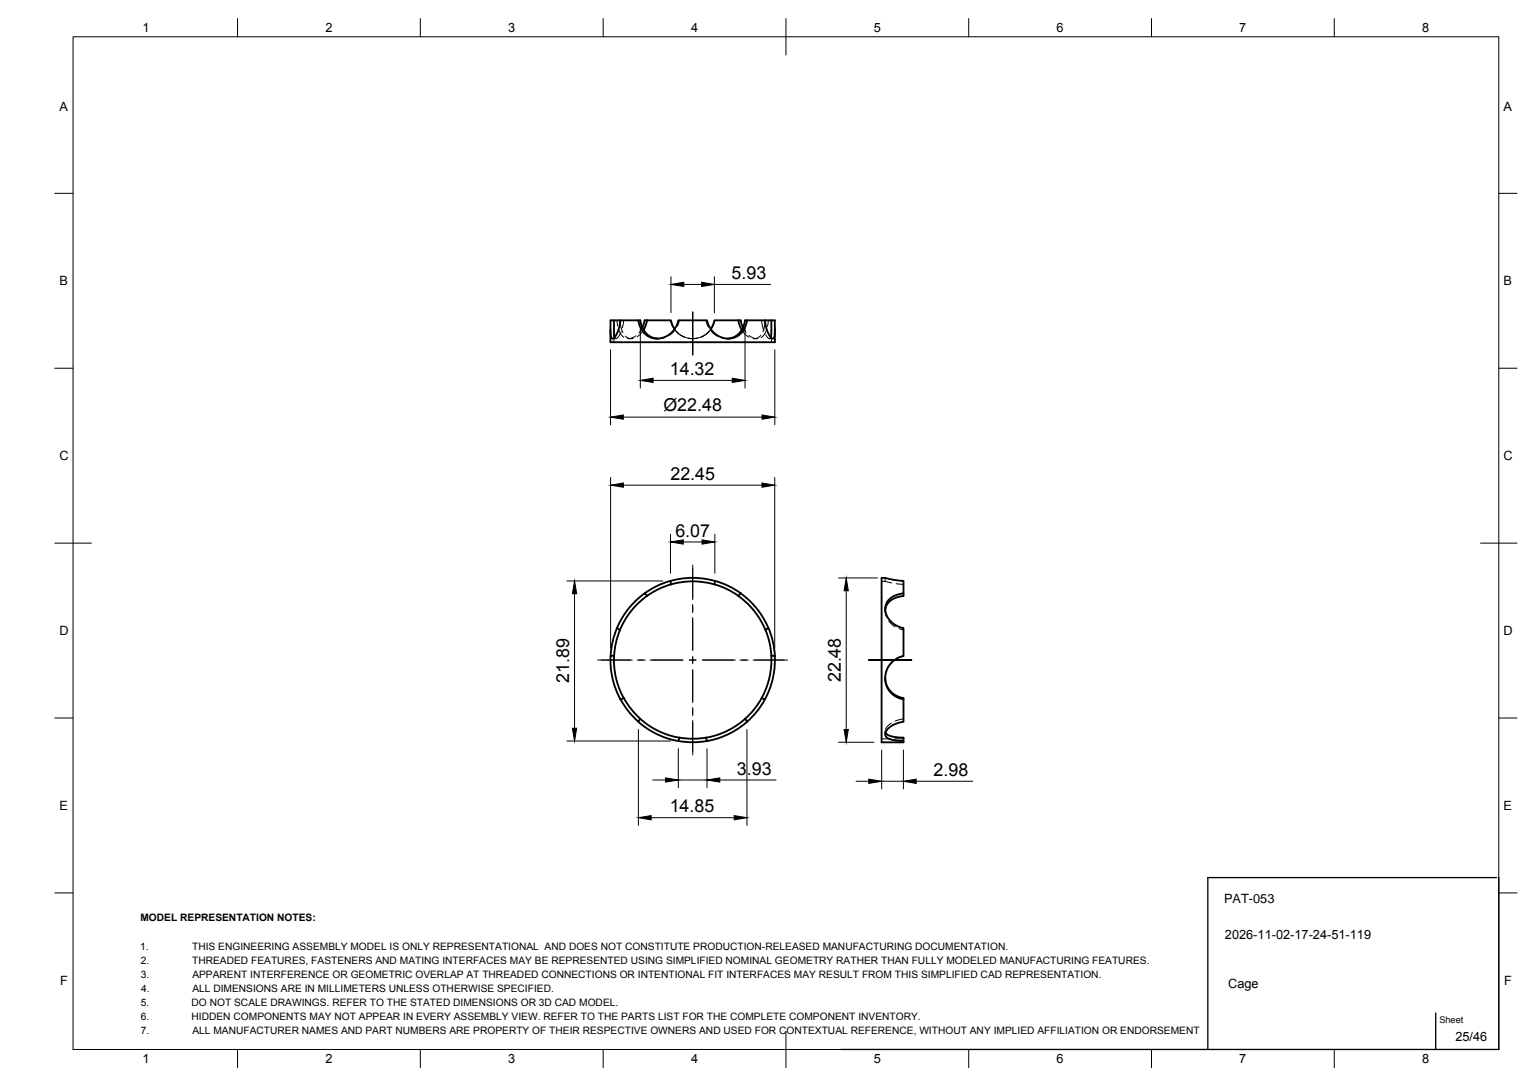
ISO-10303-21;
HEADER;
/* Generated by software containing ST-Developer
 * from STEP Tools, Inc. (www.steptools.com) 
 */

FILE_DESCRIPTION(
/* description */ ('Hand-operated arbor press'),
/* implementation_level */ '2;1');

FILE_NAME(
/* name */ 'Cage.step',
/* time_stamp */ '2026-10-28T03:25:25-07:00',
/* author */ (''),
/* organization */ (''),
/* preprocessor_version */ 'ST-DEVELOPER v20.2',
/* originating_system */ 'Autodesk Translation Framework v15.17.0.0',
/* authorisation */ '');

FILE_SCHEMA (('AUTOMOTIVE_DESIGN { 1 0 10303 214 3 1 1 }'));
ENDSEC;

DATA;
#10=MECHANICAL_DESIGN_GEOMETRIC_PRESENTATION_REPRESENTATION('',(#611),#32751);
#439=B_SPLINE_CURVE_WITH_KNOTS('',3,(#18826,#18827,#18828,#18829,#18830,
#18831,#18832,#18833,#18834,#18835,#18836,#18837,#18838,#18839,#18840,#18841,
#18842,#18843,#18844,#18845,#18846,#18847),.UNSPECIFIED.,.F.,.F.,(4,2,2,
2,2,2,2,2,2,2,4),(0.0591825211272536,0.157966726598481,0.236950089897721,
0.315933453196962,0.391576304923761,0.46721915665056,0.54286200837736,0.618504860104159,
0.697488223403399,0.77647158670264,0.875255792173867),.UNSPECIFIED.);
#440=B_SPLINE_CURVE_WITH_KNOTS('',3,(#18851,#18852,#18853,#18854,#18855,
#18856,#18857,#18858,#18859,#18860,#18861,#18862,#18863,#18864,#18865,#18866,
#18867,#18868,#18869,#18870,#18871,#18872),.UNSPECIFIED.,.F.,.F.,(4,2,2,
2,2,2,2,2,2,2,4),(0.0581119756758434,0.106553146291161,0.213106292582322,
0.30849933801665,0.386091982889075,0.4636846277615,0.541277272633925,0.61886991750635,
0.714262962940678,0.820816109231839,0.869257279847157),.UNSPECIFIED.);
#441=B_SPLINE_CURVE_WITH_KNOTS('',3,(#18878,#18879,#18880,#18881,#18882,
#18883,#18884,#18885,#18886,#18887,#18888,#18889,#18890,#18891,#18892,#18893,
#18894,#18895,#18896,#18897,#18898,#18899),.UNSPECIFIED.,.F.,.F.,(4,2,2,
2,2,2,2,2,2,2,4),(0.0581119756758434,0.106553146291161,0.213106292582322,
0.30849933801665,0.386091982889075,0.4636846277615,0.541277272633925,0.61886991750635,
0.714262962940679,0.820816109231839,0.869257279847157),.UNSPECIFIED.);
#442=B_SPLINE_CURVE_WITH_KNOTS('',3,(#18903,#18904,#18905,#18906,#18907,
#18908,#18909,#18910,#18911,#18912,#18913,#18914,#18915,#18916,#18917,#18918,
#18919,#18920,#18921,#18922,#18923,#18924),.UNSPECIFIED.,.F.,.F.,(4,2,2,
2,2,2,2,2,2,2,4),(0.0581119756758433,0.106553146291161,0.213106292582322,
0.308499338016649,0.386091982889075,0.4636846277615,0.541277272633925,0.61886991750635,
0.714262962940678,0.820816109231839,0.869257279847157),.UNSPECIFIED.);
#443=B_SPLINE_CURVE_WITH_KNOTS('',3,(#18933,#18934,#18935,#18936,#18937,
#18938,#18939,#18940,#18941,#18942,#18943,#18944,#18945,#18946,#18947,#18948,
#18949,#18950,#18951,#18952,#18953,#18954),.UNSPECIFIED.,.F.,.F.,(4,2,2,
2,2,2,2,2,2,2,4),(0.0581119756758433,0.106553146291161,0.213106292582322,
0.30849933801665,0.386091982889075,0.4636846277615,0.541277272633925,0.61886991750635,
0.714262962940678,0.820816109231839,0.869257279847157),.UNSPECIFIED.);
#444=B_SPLINE_CURVE_WITH_KNOTS('',3,(#18958,#18959,#18960,#18961,#18962,
#18963,#18964,#18965,#18966,#18967,#18968,#18969,#18970,#18971,#18972,#18973,
#18974,#18975,#18976,#18977,#18978,#18979),.UNSPECIFIED.,.F.,.F.,(4,2,2,
2,2,2,2,2,2,2,4),(0.0581119756758434,0.106553146291161,0.213106292582322,
0.30849933801665,0.386091982889075,0.4636846277615,0.541277272633925,0.61886991750635,
0.714262962940678,0.820816109231839,0.869257279847157),.UNSPECIFIED.);
#445=B_SPLINE_CURVE_WITH_KNOTS('',3,(#18983,#18984,#18985,#18986,#18987,
#18988,#18989,#18990,#18991,#18992,#18993,#18994,#18995,#18996,#18997,#18998,
#18999,#19000,#19001,#19002,#19003,#19004),.UNSPECIFIED.,.F.,.F.,(4,2,2,
2,2,2,2,2,2,2,4),(0.0581119756758434,0.106553146291161,0.213106292582322,
0.30849933801665,0.386091982889075,0.4636846277615,0.541277272633925,0.61886991750635,
0.714262962940678,0.820816109231839,0.869257279847157),.UNSPECIFIED.);
#446=B_SPLINE_CURVE_WITH_KNOTS('',3,(#19008,#19009,#19010,#19011,#19012,
#19013,#19014,#19015,#19016,#19017,#19018,#19019,#19020,#19021,#19022,#19023,
#19024,#19025,#19026,#19027,#19028,#19029),.UNSPECIFIED.,.F.,.F.,(4,2,2,
2,2,2,2,2,2,2,4),(0.0581119756758433,0.106553146291161,0.213106292582322,
0.30849933801665,0.386091982889075,0.4636846277615,0.541277272633925,0.61886991750635,
0.714262962940678,0.820816109231839,0.869257279847157),.UNSPECIFIED.);
#447=B_SPLINE_CURVE_WITH_KNOTS('',3,(#19037,#19038,#19039,#19040,#19041,
#19042,#19043,#19044,#19045,#19046,#19047,#19048,#19049,#19050,#19051,#19052,
#19053,#19054,#19055,#19056,#19057,#19058),.UNSPECIFIED.,.F.,.F.,(4,2,2,
2,2,2,2,2,2,2,4),(0.0591825211272536,0.157966726598481,0.236950089897721,
0.315933453196962,0.391576304923761,0.467219156650561,0.54286200837736,
0.618504860104159,0.697488223403399,0.77647158670264,0.875255792173867),
 .UNSPECIFIED.);
#448=B_SPLINE_CURVE_WITH_KNOTS('',3,(#19066,#19067,#19068,#19069,#19070,
#19071,#19072,#19073,#19074,#19075,#19076,#19077,#19078,#19079,#19080,#19081,
#19082,#19083,#19084,#19085,#19086,#19087),.UNSPECIFIED.,.F.,.F.,(4,2,2,
2,2,2,2,2,2,2,4),(0.0591825211272536,0.157966726598481,0.236950089897722,
0.315933453196962,0.391576304923761,0.467219156650561,0.54286200837736,
0.618504860104159,0.697488223403399,0.77647158670264,0.875255792173867),
 .UNSPECIFIED.);
#449=B_SPLINE_CURVE_WITH_KNOTS('',3,(#19097,#19098,#19099,#19100,#19101,
#19102,#19103,#19104,#19105,#19106,#19107,#19108,#19109,#19110,#19111,#19112,
#19113,#19114,#19115,#19116,#19117,#19118),.UNSPECIFIED.,.F.,.F.,(4,2,2,
2,2,2,2,2,2,2,4),(0.0591825211272536,0.157966726598481,0.236950089897721,
0.315933453196962,0.391576304923761,0.46721915665056,0.54286200837736,0.618504860104159,
0.697488223403399,0.77647158670264,0.875255792173867),.UNSPECIFIED.);
#450=B_SPLINE_CURVE_WITH_KNOTS('',3,(#19126,#19127,#19128,#19129,#19130,
#19131,#19132,#19133,#19134,#19135,#19136,#19137,#19138,#19139,#19140,#19141,
#19142,#19143,#19144,#19145,#19146,#19147),.UNSPECIFIED.,.F.,.F.,(4,2,2,
2,2,2,2,2,2,2,4),(0.0591825211272536,0.157966726598481,0.236950089897721,
0.315933453196962,0.391576304923761,0.46721915665056,0.542862008377359,
0.618504860104159,0.697488223403399,0.776471586702639,0.875255792173867),
 .UNSPECIFIED.);
#451=B_SPLINE_CURVE_WITH_KNOTS('',3,(#19155,#19156,#19157,#19158,#19159,
#19160,#19161,#19162,#19163,#19164,#19165,#19166,#19167,#19168,#19169,#19170,
#19171,#19172,#19173,#19174,#19175,#19176),.UNSPECIFIED.,.F.,.F.,(4,2,2,
2,2,2,2,2,2,2,4),(0.0591825211272536,0.157966726598481,0.236950089897721,
0.315933453196962,0.391576304923761,0.46721915665056,0.54286200837736,0.618504860104159,
0.697488223403399,0.77647158670264,0.875255792173867),.UNSPECIFIED.);
#452=B_SPLINE_CURVE_WITH_KNOTS('',3,(#19185,#19186,#19187,#19188,#19189,
#19190,#19191,#19192,#19193,#19194,#19195,#19196,#19197,#19198,#19199,#19200,
#19201,#19202,#19203,#19204,#19205,#19206),.UNSPECIFIED.,.F.,.F.,(4,2,2,
2,2,2,2,2,2,2,4),(0.0591825211272536,0.157966726598481,0.236950089897721,
0.315933453196962,0.391576304923761,0.46721915665056,0.542862008377359,
0.618504860104159,0.697488223403399,0.776471586702639,0.875255792173867),
 .UNSPECIFIED.);
#464=SPHERICAL_SURFACE('',#13471,0.309556);
#465=SPHERICAL_SURFACE('',#13487,0.309556);
#466=SPHERICAL_SURFACE('',#13492,0.309556);
#467=SPHERICAL_SURFACE('',#13498,0.309556);
#468=SPHERICAL_SURFACE('',#13503,0.309556);
#469=SPHERICAL_SURFACE('',#13508,0.309556);
#470=SPHERICAL_SURFACE('',#13516,0.309556);
#521=SHAPE_REPRESENTATION_RELATIONSHIP('SRR','None',#32951,#563);
#563=ADVANCED_BREP_SHAPE_REPRESENTATION('',(#659),#32725);
#611=STYLED_ITEM('',(#33242),#659);
#659=MANIFOLD_SOLID_BREP('Continuous crown cage',#12509);
#806=FACE_BOUND('',#2358,.T.);
#981=PLANE('',#13484);
#982=PLANE('',#13489);
#983=PLANE('',#13494);
#984=PLANE('',#13500);
#985=PLANE('',#13505);
#986=PLANE('',#13514);
#987=PLANE('',#13518);
#988=PLANE('',#13519);
#1535=FACE_OUTER_BOUND('',#2342,.T.);
#1536=FACE_OUTER_BOUND('',#2343,.T.);
#1537=FACE_OUTER_BOUND('',#2344,.T.);
#1538=FACE_OUTER_BOUND('',#2345,.T.);
#1539=FACE_OUTER_BOUND('',#2346,.T.);
#1540=FACE_OUTER_BOUND('',#2347,.T.);
#1541=FACE_OUTER_BOUND('',#2348,.T.);
#1542=FACE_OUTER_BOUND('',#2349,.T.);
#1543=FACE_OUTER_BOUND('',#2350,.T.);
#1544=FACE_OUTER_BOUND('',#2351,.T.);
#1545=FACE_OUTER_BOUND('',#2352,.T.);
#1546=FACE_OUTER_BOUND('',#2353,.T.);
#1547=FACE_OUTER_BOUND('',#2354,.T.);
#1548=FACE_OUTER_BOUND('',#2355,.T.);
#1549=FACE_OUTER_BOUND('',#2356,.T.);
#1550=FACE_OUTER_BOUND('',#2357,.T.);
#1551=FACE_OUTER_BOUND('',#2359,.T.);
#2342=EDGE_LOOP('',(#9420,#9421,#9422,#9423));
#2343=EDGE_LOOP('',(#9424,#9425,#9426,#9427,#9428,#9429,#9430,#9431,#9432,
#9433,#9434,#9435,#9436,#9437,#9438,#9439,#9440,#9441));
#2344=EDGE_LOOP('',(#9442,#9443,#9444,#9445));
#2345=EDGE_LOOP('',(#9446,#9447,#9448,#9449));
#2346=EDGE_LOOP('',(#9450,#9451,#9452,#9453));
#2347=EDGE_LOOP('',(#9454,#9455,#9456,#9457));
#2348=EDGE_LOOP('',(#9458,#9459,#9460,#9461,#9462,#9463));
#2349=EDGE_LOOP('',(#9464,#9465,#9466,#9467));
#2350=EDGE_LOOP('',(#9468,#9469,#9470,#9471));
#2351=EDGE_LOOP('',(#9472,#9473,#9474,#9475));
#2352=EDGE_LOOP('',(#9476,#9477,#9478,#9479));
#2353=EDGE_LOOP('',(#9480,#9481,#9482,#9483));
#2354=EDGE_LOOP('',(#9484,#9485,#9486,#9487,#9488,#9489,#9490,#9491,#9492,
#9493,#9494,#9495,#9496,#9497,#9498,#9499,#9500,#9501));
#2355=EDGE_LOOP('',(#9502,#9503,#9504,#9505));
#2356=EDGE_LOOP('',(#9506,#9507,#9508,#9509));
#2357=EDGE_LOOP('',(#9510));
#2358=EDGE_LOOP('',(#9511));
#2359=EDGE_LOOP('',(#9512,#9513,#9514,#9515));
#3165=LINE('',#18928,#4336);
#3166=LINE('',#19181,#4337);
#4336=VECTOR('',#15454,1.123812);
#4337=VECTOR('',#15523,1.076188);
#5373=CIRCLE('',#13472,0.303778037777585);
#5374=CIRCLE('',#13473,0.303778037777585);
#5375=CIRCLE('',#13475,1.123812);
#5376=CIRCLE('',#13476,1.123812);
#5377=CIRCLE('',#13477,1.123812);
#5378=CIRCLE('',#13478,1.123812);
#5379=CIRCLE('',#13479,1.123812);
#5380=CIRCLE('',#13480,1.123812);
#5381=CIRCLE('',#13481,1.123812);
#5382=CIRCLE('',#13482,1.123812);
#5383=CIRCLE('',#13483,1.123812);
#5384=CIRCLE('',#13485,1.076188);
#5385=CIRCLE('',#13486,0.303778037777585);
#5386=CIRCLE('',#13488,0.303778037777585);
#5387=CIRCLE('',#13490,1.076188);
#5388=CIRCLE('',#13491,0.303778037777585);
#5389=CIRCLE('',#13493,0.303778037777585);
#5390=CIRCLE('',#13495,1.076188);
#5391=CIRCLE('',#13496,1.076188);
#5392=CIRCLE('',#13497,0.303778037777585);
#5393=CIRCLE('',#13499,0.303778037777585);
#5394=CIRCLE('',#13501,1.076188);
#5395=CIRCLE('',#13502,0.303778037777585);
#5396=CIRCLE('',#13504,0.303778037777585);
#5397=CIRCLE('',#13506,1.076188);
#5398=CIRCLE('',#13507,0.303778037777585);
#5399=CIRCLE('',#13509,0.303778037777585);
#5400=CIRCLE('',#13511,1.076188);
#5401=CIRCLE('',#13512,1.076188);
#5402=CIRCLE('',#13513,1.076188);
#5403=CIRCLE('',#13515,0.303778037777585);
#5404=CIRCLE('',#13517,0.303778037777585);
#5928=VERTEX_POINT('',#18824);
#5929=VERTEX_POINT('',#18825);
#5930=VERTEX_POINT('',#18848);
#5931=VERTEX_POINT('',#18850);
#5932=VERTEX_POINT('',#18875);
#5933=VERTEX_POINT('',#18877);
#5934=VERTEX_POINT('',#18900);
#5935=VERTEX_POINT('',#18902);
#5936=VERTEX_POINT('',#18925);
#5937=VERTEX_POINT('',#18927);
#5938=VERTEX_POINT('',#18930);
#5939=VERTEX_POINT('',#18932);
#5940=VERTEX_POINT('',#18955);
#5941=VERTEX_POINT('',#18957);
#5942=VERTEX_POINT('',#18980);
#5943=VERTEX_POINT('',#18982);
#5944=VERTEX_POINT('',#19005);
#5945=VERTEX_POINT('',#19007);
#5946=VERTEX_POINT('',#19032);
#5947=VERTEX_POINT('',#19036);
#5948=VERTEX_POINT('',#19061);
#5949=VERTEX_POINT('',#19065);
#5950=VERTEX_POINT('',#19090);
#5951=VERTEX_POINT('',#19092);
#5952=VERTEX_POINT('',#19096);
#5953=VERTEX_POINT('',#19121);
#5954=VERTEX_POINT('',#19125);
#5955=VERTEX_POINT('',#19150);
#5956=VERTEX_POINT('',#19154);
#5957=VERTEX_POINT('',#19179);
#5958=VERTEX_POINT('',#19182);
#5959=VERTEX_POINT('',#19184);
#7213=EDGE_CURVE('',#5928,#5929,#439,.T.);
#7214=EDGE_CURVE('',#5930,#5928,#5373,.T.);
#7215=EDGE_CURVE('',#5931,#5930,#440,.T.);
#7216=EDGE_CURVE('',#5929,#5931,#5374,.T.);
#7217=EDGE_CURVE('',#5932,#5930,#5375,.T.);
#7218=EDGE_CURVE('',#5932,#5933,#441,.T.);
#7219=EDGE_CURVE('',#5934,#5933,#5376,.T.);
#7220=EDGE_CURVE('',#5934,#5935,#442,.T.);
#7221=EDGE_CURVE('',#5936,#5935,#5377,.T.);
#7222=EDGE_CURVE('',#5936,#5937,#3165,.T.);
#7223=EDGE_CURVE('',#5937,#5937,#5378,.T.);
#7224=EDGE_CURVE('',#5938,#5936,#5379,.T.);
#7225=EDGE_CURVE('',#5938,#5939,#443,.T.);
#7226=EDGE_CURVE('',#5940,#5939,#5380,.T.);
#7227=EDGE_CURVE('',#5940,#5941,#444,.T.);
#7228=EDGE_CURVE('',#5942,#5941,#5381,.T.);
#7229=EDGE_CURVE('',#5942,#5943,#445,.T.);
#7230=EDGE_CURVE('',#5944,#5943,#5382,.T.);
#7231=EDGE_CURVE('',#5944,#5945,#446,.T.);
#7232=EDGE_CURVE('',#5931,#5945,#5383,.T.);
#7233=EDGE_CURVE('',#5928,#5946,#5384,.T.);
#7234=EDGE_CURVE('',#5946,#5932,#5385,.T.);
#7235=EDGE_CURVE('',#5947,#5946,#447,.T.);
#7236=EDGE_CURVE('',#5933,#5947,#5386,.T.);
#7237=EDGE_CURVE('',#5947,#5948,#5387,.T.);
#7238=EDGE_CURVE('',#5948,#5934,#5388,.T.);
#7239=EDGE_CURVE('',#5949,#5948,#448,.T.);
#7240=EDGE_CURVE('',#5935,#5949,#5389,.T.);
#7241=EDGE_CURVE('',#5949,#5950,#5390,.T.);
#7242=EDGE_CURVE('',#5950,#5951,#5391,.T.);
#7243=EDGE_CURVE('',#5951,#5938,#5392,.T.);
#7244=EDGE_CURVE('',#5952,#5951,#449,.T.);
#7245=EDGE_CURVE('',#5939,#5952,#5393,.T.);
#7246=EDGE_CURVE('',#5952,#5953,#5394,.T.);
#7247=EDGE_CURVE('',#5953,#5940,#5395,.T.);
#7248=EDGE_CURVE('',#5954,#5953,#450,.T.);
#7249=EDGE_CURVE('',#5941,#5954,#5396,.T.);
#7250=EDGE_CURVE('',#5954,#5955,#5397,.T.);
#7251=EDGE_CURVE('',#5955,#5942,#5398,.T.);
#7252=EDGE_CURVE('',#5956,#5955,#451,.T.);
#7253=EDGE_CURVE('',#5943,#5956,#5399,.T.);
#7254=EDGE_CURVE('',#5957,#5957,#5400,.T.);
#7255=EDGE_CURVE('',#5957,#5950,#3166,.T.);
#7256=EDGE_CURVE('',#5958,#5929,#5401,.T.);
#7257=EDGE_CURVE('',#5958,#5959,#452,.T.);
#7258=EDGE_CURVE('',#5956,#5959,#5402,.T.);
#7259=EDGE_CURVE('',#5945,#5958,#5403,.T.);
#7260=EDGE_CURVE('',#5959,#5944,#5404,.T.);
#9420=ORIENTED_EDGE('',*,*,#7213,.F.);
#9421=ORIENTED_EDGE('',*,*,#7214,.F.);
#9422=ORIENTED_EDGE('',*,*,#7215,.F.);
#9423=ORIENTED_EDGE('',*,*,#7216,.F.);
#9424=ORIENTED_EDGE('',*,*,#7215,.T.);
#9425=ORIENTED_EDGE('',*,*,#7217,.F.);
#9426=ORIENTED_EDGE('',*,*,#7218,.T.);
#9427=ORIENTED_EDGE('',*,*,#7219,.F.);
#9428=ORIENTED_EDGE('',*,*,#7220,.T.);
#9429=ORIENTED_EDGE('',*,*,#7221,.F.);
#9430=ORIENTED_EDGE('',*,*,#7222,.T.);
#9431=ORIENTED_EDGE('',*,*,#7223,.F.);
#9432=ORIENTED_EDGE('',*,*,#7222,.F.);
#9433=ORIENTED_EDGE('',*,*,#7224,.F.);
#9434=ORIENTED_EDGE('',*,*,#7225,.T.);
#9435=ORIENTED_EDGE('',*,*,#7226,.F.);
#9436=ORIENTED_EDGE('',*,*,#7227,.T.);
#9437=ORIENTED_EDGE('',*,*,#7228,.F.);
#9438=ORIENTED_EDGE('',*,*,#7229,.T.);
#9439=ORIENTED_EDGE('',*,*,#7230,.F.);
#9440=ORIENTED_EDGE('',*,*,#7231,.T.);
#9441=ORIENTED_EDGE('',*,*,#7232,.F.);
#9442=ORIENTED_EDGE('',*,*,#7214,.T.);
#9443=ORIENTED_EDGE('',*,*,#7233,.T.);
#9444=ORIENTED_EDGE('',*,*,#7234,.T.);
#9445=ORIENTED_EDGE('',*,*,#7217,.T.);
#9446=ORIENTED_EDGE('',*,*,#7235,.F.);
#9447=ORIENTED_EDGE('',*,*,#7236,.F.);
#9448=ORIENTED_EDGE('',*,*,#7218,.F.);
#9449=ORIENTED_EDGE('',*,*,#7234,.F.);
#9450=ORIENTED_EDGE('',*,*,#7236,.T.);
#9451=ORIENTED_EDGE('',*,*,#7237,.T.);
#9452=ORIENTED_EDGE('',*,*,#7238,.T.);
#9453=ORIENTED_EDGE('',*,*,#7219,.T.);
#9454=ORIENTED_EDGE('',*,*,#7239,.F.);
#9455=ORIENTED_EDGE('',*,*,#7240,.F.);
#9456=ORIENTED_EDGE('',*,*,#7220,.F.);
#9457=ORIENTED_EDGE('',*,*,#7238,.F.);
#9458=ORIENTED_EDGE('',*,*,#7240,.T.);
#9459=ORIENTED_EDGE('',*,*,#7241,.T.);
#9460=ORIENTED_EDGE('',*,*,#7242,.T.);
#9461=ORIENTED_EDGE('',*,*,#7243,.T.);
#9462=ORIENTED_EDGE('',*,*,#7224,.T.);
#9463=ORIENTED_EDGE('',*,*,#7221,.T.);
#9464=ORIENTED_EDGE('',*,*,#7244,.F.);
#9465=ORIENTED_EDGE('',*,*,#7245,.F.);
#9466=ORIENTED_EDGE('',*,*,#7225,.F.);
#9467=ORIENTED_EDGE('',*,*,#7243,.F.);
#9468=ORIENTED_EDGE('',*,*,#7245,.T.);
#9469=ORIENTED_EDGE('',*,*,#7246,.T.);
#9470=ORIENTED_EDGE('',*,*,#7247,.T.);
#9471=ORIENTED_EDGE('',*,*,#7226,.T.);
#9472=ORIENTED_EDGE('',*,*,#7248,.F.);
#9473=ORIENTED_EDGE('',*,*,#7249,.F.);
#9474=ORIENTED_EDGE('',*,*,#7227,.F.);
#9475=ORIENTED_EDGE('',*,*,#7247,.F.);
#9476=ORIENTED_EDGE('',*,*,#7249,.T.);
#9477=ORIENTED_EDGE('',*,*,#7250,.T.);
#9478=ORIENTED_EDGE('',*,*,#7251,.T.);
#9479=ORIENTED_EDGE('',*,*,#7228,.T.);
#9480=ORIENTED_EDGE('',*,*,#7229,.F.);
#9481=ORIENTED_EDGE('',*,*,#7251,.F.);
#9482=ORIENTED_EDGE('',*,*,#7252,.F.);
#9483=ORIENTED_EDGE('',*,*,#7253,.F.);
#9484=ORIENTED_EDGE('',*,*,#7254,.F.);
#9485=ORIENTED_EDGE('',*,*,#7255,.T.);
#9486=ORIENTED_EDGE('',*,*,#7241,.F.);
#9487=ORIENTED_EDGE('',*,*,#7239,.T.);
#9488=ORIENTED_EDGE('',*,*,#7237,.F.);
#9489=ORIENTED_EDGE('',*,*,#7235,.T.);
#9490=ORIENTED_EDGE('',*,*,#7233,.F.);
#9491=ORIENTED_EDGE('',*,*,#7213,.T.);
#9492=ORIENTED_EDGE('',*,*,#7256,.F.);
#9493=ORIENTED_EDGE('',*,*,#7257,.T.);
#9494=ORIENTED_EDGE('',*,*,#7258,.F.);
#9495=ORIENTED_EDGE('',*,*,#7252,.T.);
#9496=ORIENTED_EDGE('',*,*,#7250,.F.);
#9497=ORIENTED_EDGE('',*,*,#7248,.T.);
#9498=ORIENTED_EDGE('',*,*,#7246,.F.);
#9499=ORIENTED_EDGE('',*,*,#7244,.T.);
#9500=ORIENTED_EDGE('',*,*,#7242,.F.);
#9501=ORIENTED_EDGE('',*,*,#7255,.F.);
#9502=ORIENTED_EDGE('',*,*,#7216,.T.);
#9503=ORIENTED_EDGE('',*,*,#7232,.T.);
#9504=ORIENTED_EDGE('',*,*,#7259,.T.);
#9505=ORIENTED_EDGE('',*,*,#7256,.T.);
#9506=ORIENTED_EDGE('',*,*,#7231,.F.);
#9507=ORIENTED_EDGE('',*,*,#7260,.F.);
#9508=ORIENTED_EDGE('',*,*,#7257,.F.);
#9509=ORIENTED_EDGE('',*,*,#7259,.F.);
#9510=ORIENTED_EDGE('',*,*,#7223,.T.);
#9511=ORIENTED_EDGE('',*,*,#7254,.T.);
#9512=ORIENTED_EDGE('',*,*,#7253,.T.);
#9513=ORIENTED_EDGE('',*,*,#7258,.T.);
#9514=ORIENTED_EDGE('',*,*,#7260,.T.);
#9515=ORIENTED_EDGE('',*,*,#7230,.T.);
#11735=CYLINDRICAL_SURFACE('',#13474,1.123812);
#11736=CYLINDRICAL_SURFACE('',#13510,1.076188);
#12044=ADVANCED_FACE('',(#1535),#464,.F.);
#12045=ADVANCED_FACE('',(#1536),#11735,.T.);
#12046=ADVANCED_FACE('',(#1537),#981,.T.);
#12047=ADVANCED_FACE('',(#1538),#465,.F.);
#12048=ADVANCED_FACE('',(#1539),#982,.T.);
#12049=ADVANCED_FACE('',(#1540),#466,.F.);
#12050=ADVANCED_FACE('',(#1541),#983,.T.);
#12051=ADVANCED_FACE('',(#1542),#467,.F.);
#12052=ADVANCED_FACE('',(#1543),#984,.T.);
#12053=ADVANCED_FACE('',(#1544),#468,.F.);
#12054=ADVANCED_FACE('',(#1545),#985,.T.);
#12055=ADVANCED_FACE('',(#1546),#469,.F.);
#12056=ADVANCED_FACE('',(#1547),#11736,.F.);
#12057=ADVANCED_FACE('',(#1548),#986,.T.);
#12058=ADVANCED_FACE('',(#1549),#470,.F.);
#12059=ADVANCED_FACE('',(#1550,#806),#987,.T.);
#12060=ADVANCED_FACE('',(#1551),#988,.T.);
#12509=CLOSED_SHELL('',(#12044,#12045,#12046,#12047,#12048,#12049,#12050,
#12051,#12052,#12053,#12054,#12055,#12056,#12057,#12058,#12059,#12060));
#13470=AXIS2_PLACEMENT_3D('',#18822,#15438,#15439);
#13471=AXIS2_PLACEMENT_3D('',#18823,#15440,#15441);
#13472=AXIS2_PLACEMENT_3D('',#18849,#15442,#15443);
#13473=AXIS2_PLACEMENT_3D('',#18873,#15444,#15445);
#13474=AXIS2_PLACEMENT_3D('',#18874,#15446,#15447);
#13475=AXIS2_PLACEMENT_3D('',#18876,#15448,#15449);
#13476=AXIS2_PLACEMENT_3D('',#18901,#15450,#15451);
#13477=AXIS2_PLACEMENT_3D('',#18926,#15452,#15453);
#13478=AXIS2_PLACEMENT_3D('',#18929,#15455,#15456);
#13479=AXIS2_PLACEMENT_3D('',#18931,#15457,#15458);
#13480=AXIS2_PLACEMENT_3D('',#18956,#15459,#15460);
#13481=AXIS2_PLACEMENT_3D('',#18981,#15461,#15462);
#13482=AXIS2_PLACEMENT_3D('',#19006,#15463,#15464);
#13483=AXIS2_PLACEMENT_3D('',#19030,#15465,#15466);
#13484=AXIS2_PLACEMENT_3D('',#19031,#15467,#15468);
#13485=AXIS2_PLACEMENT_3D('',#19033,#15469,#15470);
#13486=AXIS2_PLACEMENT_3D('',#19034,#15471,#15472);
#13487=AXIS2_PLACEMENT_3D('',#19035,#15473,#15474);
#13488=AXIS2_PLACEMENT_3D('',#19059,#15475,#15476);
#13489=AXIS2_PLACEMENT_3D('',#19060,#15477,#15478);
#13490=AXIS2_PLACEMENT_3D('',#19062,#15479,#15480);
#13491=AXIS2_PLACEMENT_3D('',#19063,#15481,#15482);
#13492=AXIS2_PLACEMENT_3D('',#19064,#15483,#15484);
#13493=AXIS2_PLACEMENT_3D('',#19088,#15485,#15486);
#13494=AXIS2_PLACEMENT_3D('',#19089,#15487,#15488);
#13495=AXIS2_PLACEMENT_3D('',#19091,#15489,#15490);
#13496=AXIS2_PLACEMENT_3D('',#19093,#15491,#15492);
#13497=AXIS2_PLACEMENT_3D('',#19094,#15493,#15494);
#13498=AXIS2_PLACEMENT_3D('',#19095,#15495,#15496);
#13499=AXIS2_PLACEMENT_3D('',#19119,#15497,#15498);
#13500=AXIS2_PLACEMENT_3D('',#19120,#15499,#15500);
#13501=AXIS2_PLACEMENT_3D('',#19122,#15501,#15502);
#13502=AXIS2_PLACEMENT_3D('',#19123,#15503,#15504);
#13503=AXIS2_PLACEMENT_3D('',#19124,#15505,#15506);
#13504=AXIS2_PLACEMENT_3D('',#19148,#15507,#15508);
#13505=AXIS2_PLACEMENT_3D('',#19149,#15509,#15510);
#13506=AXIS2_PLACEMENT_3D('',#19151,#15511,#15512);
#13507=AXIS2_PLACEMENT_3D('',#19152,#15513,#15514);
#13508=AXIS2_PLACEMENT_3D('',#19153,#15515,#15516);
#13509=AXIS2_PLACEMENT_3D('',#19177,#15517,#15518);
#13510=AXIS2_PLACEMENT_3D('',#19178,#15519,#15520);
#13511=AXIS2_PLACEMENT_3D('',#19180,#15521,#15522);
#13512=AXIS2_PLACEMENT_3D('',#19183,#15524,#15525);
#13513=AXIS2_PLACEMENT_3D('',#19207,#15526,#15527);
#13514=AXIS2_PLACEMENT_3D('',#19208,#15528,#15529);
#13515=AXIS2_PLACEMENT_3D('',#19209,#15530,#15531);
#13516=AXIS2_PLACEMENT_3D('',#19210,#15532,#15533);
#13517=AXIS2_PLACEMENT_3D('',#19211,#15534,#15535);
#13518=AXIS2_PLACEMENT_3D('',#19212,#15536,#15537);
#13519=AXIS2_PLACEMENT_3D('',#19213,#15538,#15539);
#15438=DIRECTION('axis',(0.,0.,1.));
#15439=DIRECTION('refdir',(1.,0.,0.));
#15440=DIRECTION('center_axis',(0.,0.,1.));
#15441=DIRECTION('ref_axis',(1.,0.,0.));
#15442=DIRECTION('center_axis',(0.,-1.,0.));
#15443=DIRECTION('ref_axis',(0.,0.,-1.));
#15444=DIRECTION('center_axis',(0.,-1.,0.));
#15445=DIRECTION('ref_axis',(0.,0.,-1.));
#15446=DIRECTION('center_axis',(0.,1.,0.));
#15447=DIRECTION('ref_axis',(1.,0.,0.));
#15448=DIRECTION('center_axis',(0.,1.,0.));
#15449=DIRECTION('ref_axis',(1.,0.,0.));
#15450=DIRECTION('center_axis',(0.,1.,0.));
#15451=DIRECTION('ref_axis',(1.,0.,0.));
#15452=DIRECTION('center_axis',(0.,1.,0.));
#15453=DIRECTION('ref_axis',(1.,0.,0.));
#15454=DIRECTION('',(0.,-1.,0.));
#15455=DIRECTION('center_axis',(0.,-1.,0.));
#15456=DIRECTION('ref_axis',(1.,0.,0.));
#15457=DIRECTION('center_axis',(0.,1.,0.));
#15458=DIRECTION('ref_axis',(1.,0.,0.));
#15459=DIRECTION('center_axis',(0.,1.,0.));
#15460=DIRECTION('ref_axis',(1.,0.,0.));
#15461=DIRECTION('center_axis',(0.,1.,0.));
#15462=DIRECTION('ref_axis',(1.,0.,0.));
#15463=DIRECTION('center_axis',(0.,1.,0.));
#15464=DIRECTION('ref_axis',(1.,0.,0.));
#15465=DIRECTION('center_axis',(0.,1.,0.));
#15466=DIRECTION('ref_axis',(1.,0.,0.));
#15467=DIRECTION('center_axis',(0.,1.,0.));
#15468=DIRECTION('ref_axis',(1.,0.,0.));
#15469=DIRECTION('center_axis',(0.,-1.,0.));
#15470=DIRECTION('ref_axis',(1.,0.,0.));
#15471=DIRECTION('center_axis',(0.,-1.,0.));
#15472=DIRECTION('ref_axis',(0.,0.,-1.));
#15473=DIRECTION('center_axis',(8.96625347776458E-17,0.,1.));
#15474=DIRECTION('ref_axis',(1.,0.,0.));
#15475=DIRECTION('center_axis',(0.,-1.,0.));
#15476=DIRECTION('ref_axis',(0.,0.,-1.));
#15477=DIRECTION('center_axis',(0.,1.,0.));
#15478=DIRECTION('ref_axis',(1.,0.,0.));
#15479=DIRECTION('center_axis',(0.,-1.,0.));
#15480=DIRECTION('ref_axis',(1.,0.,0.));
#15481=DIRECTION('center_axis',(0.,-1.,0.));
#15482=DIRECTION('ref_axis',(0.,0.,-1.));
#15483=DIRECTION('center_axis',(0.,0.,1.));
#15484=DIRECTION('ref_axis',(1.,0.,0.));
#15485=DIRECTION('center_axis',(0.,-1.,0.));
#15486=DIRECTION('ref_axis',(0.,0.,-1.));
#15487=DIRECTION('center_axis',(0.,1.,0.));
#15488=DIRECTION('ref_axis',(1.,0.,0.));
#15489=DIRECTION('center_axis',(0.,-1.,0.));
#15490=DIRECTION('ref_axis',(1.,0.,0.));
#15491=DIRECTION('center_axis',(0.,-1.,0.));
#15492=DIRECTION('ref_axis',(1.,0.,0.));
#15493=DIRECTION('center_axis',(0.,-1.,0.));
#15494=DIRECTION('ref_axis',(0.,0.,-1.));
#15495=DIRECTION('center_axis',(0.,0.,1.));
#15496=DIRECTION('ref_axis',(1.,0.,0.));
#15497=DIRECTION('center_axis',(0.,-1.,0.));
#15498=DIRECTION('ref_axis',(0.,0.,-1.));
#15499=DIRECTION('center_axis',(0.,1.,0.));
#15500=DIRECTION('ref_axis',(1.,0.,0.));
#15501=DIRECTION('center_axis',(0.,-1.,0.));
#15502=DIRECTION('ref_axis',(1.,0.,0.));
#15503=DIRECTION('center_axis',(0.,-1.,0.));
#15504=DIRECTION('ref_axis',(0.,0.,-1.));
#15505=DIRECTION('center_axis',(8.96625347776458E-17,0.,1.));
#15506=DIRECTION('ref_axis',(1.,0.,0.));
#15507=DIRECTION('center_axis',(0.,-1.,0.));
#15508=DIRECTION('ref_axis',(0.,0.,-1.));
#15509=DIRECTION('center_axis',(0.,1.,0.));
#15510=DIRECTION('ref_axis',(1.,0.,0.));
#15511=DIRECTION('center_axis',(0.,-1.,0.));
#15512=DIRECTION('ref_axis',(1.,0.,0.));
#15513=DIRECTION('center_axis',(0.,-1.,0.));
#15514=DIRECTION('ref_axis',(0.,0.,-1.));
#15515=DIRECTION('center_axis',(0.,0.,1.));
#15516=DIRECTION('ref_axis',(1.,0.,0.));
#15517=DIRECTION('center_axis',(0.,-1.,0.));
#15518=DIRECTION('ref_axis',(0.,0.,-1.));
#15519=DIRECTION('center_axis',(0.,1.,0.));
#15520=DIRECTION('ref_axis',(1.,0.,0.));
#15521=DIRECTION('center_axis',(0.,1.,0.));
#15522=DIRECTION('ref_axis',(1.,0.,0.));
#15523=DIRECTION('',(0.,1.,0.));
#15524=DIRECTION('center_axis',(0.,-1.,0.));
#15525=DIRECTION('ref_axis',(1.,0.,0.));
#15526=DIRECTION('center_axis',(0.,-1.,0.));
#15527=DIRECTION('ref_axis',(1.,0.,0.));
#15528=DIRECTION('center_axis',(0.,1.,0.));
#15529=DIRECTION('ref_axis',(1.,0.,0.));
#15530=DIRECTION('center_axis',(0.,-1.,0.));
#15531=DIRECTION('ref_axis',(0.,0.,-1.));
#15532=DIRECTION('center_axis',(0.,0.,1.));
#15533=DIRECTION('ref_axis',(1.,0.,0.));
#15534=DIRECTION('center_axis',(0.,-1.,0.));
#15535=DIRECTION('ref_axis',(0.,0.,-1.));
#15536=DIRECTION('center_axis',(0.,-1.,0.));
#15537=DIRECTION('ref_axis',(-1.,0.,0.));
#15538=DIRECTION('center_axis',(0.,1.,0.));
#15539=DIRECTION('ref_axis',(1.,0.,0.));
#18822=CARTESIAN_POINT('',(0.,0.,0.));
#18823=CARTESIAN_POINT('Origin',(0.685838782044607,0.,0.860014630714833));
#18824=CARTESIAN_POINT('',(0.413083465285518,-0.05953,0.993751811093549));
#18825=CARTESIAN_POINT('',(0.876916659919095,-0.05953,0.623857181492959));
#18826=CARTESIAN_POINT('Ctrl Pts',(0.413083465285518,-0.05953,0.993751811093549));
#18827=CARTESIAN_POINT('Ctrl Pts',(0.419070565453383,-0.0925528133349865,
0.991263089003441));
#18828=CARTESIAN_POINT('Ctrl Pts',(0.430199341854858,-0.124911173756694,
0.986608710139579));
#18829=CARTESIAN_POINT('Ctrl Pts',(0.457978755888596,-0.177924977804098,
0.973971221090534));
#18830=CARTESIAN_POINT('Ctrl Pts',(0.473077587363685,-0.199697230012983,
0.966820759530997));
#18831=CARTESIAN_POINT('Ctrl Pts',(0.507057380724533,-0.237895043532788,
0.949440676105255));
#18832=CARTESIAN_POINT('Ctrl Pts',(0.525933334162555,-0.254319232363049,
0.939198248544428));
#18833=CARTESIAN_POINT('Ctrl Pts',(0.564362943424238,-0.28018331644634,
0.916597376014514));
#18834=CARTESIAN_POINT('Ctrl Pts',(0.585840553788742,-0.29104845371857,
0.903141581680914));
#18835=CARTESIAN_POINT('Ctrl Pts',(0.629305439856167,-0.30527573347708,
0.873412008702649));
#18836=CARTESIAN_POINT('Ctrl Pts',(0.651278921914856,-0.308638795020976,
0.857118508332695));
#18837=CARTESIAN_POINT('Ctrl Pts',(0.690705563850638,-0.308638795020976,
0.825676810575914));
#18838=CARTESIAN_POINT('Ctrl Pts',(0.711480111898423,-0.30527573347708,
0.807879894508811));
#18839=CARTESIAN_POINT('Ctrl Pts',(0.750136149454208,-0.29104845371857,
0.772120216227122));
#18840=CARTESIAN_POINT('Ctrl Pts',(0.768033796848072,-0.28018331644634,
0.754175290318038));
#18841=CARTESIAN_POINT('Ctrl Pts',(0.798619410861634,-0.254319232363049,
0.721738358858166));
#18842=CARTESIAN_POINT('Ctrl Pts',(0.812805334167529,-0.237895043532788,
0.705614819529209));
#18843=CARTESIAN_POINT('Ctrl Pts',(0.837310877969633,-0.199697230012983,
0.676354402927683));
#18844=CARTESIAN_POINT('Ctrl Pts',(0.847641868610495,-0.177924977804098,
0.663225258065736));
#18845=CARTESIAN_POINT('Ctrl Pts',(0.866144010579847,-0.124911173756694,
0.638954437806245));
#18846=CARTESIAN_POINT('Ctrl Pts',(0.873158080166742,-0.0925528133349865,
0.62914037979579));
#18847=CARTESIAN_POINT('Ctrl Pts',(0.876916659919095,-0.05953,0.623857181492959));
#18848=CARTESIAN_POINT('',(0.437601487681057,-0.05953,1.03511272300331));
#18849=CARTESIAN_POINT('Origin',(0.685838782044607,-0.05953,0.860014630714833));
#18850=CARTESIAN_POINT('',(0.911784794170997,-0.05953,0.656964154625313));
#18851=CARTESIAN_POINT('Ctrl Pts',(0.911784794170998,-0.0595300000000001,
0.656964154625312));
#18852=CARTESIAN_POINT('Ctrl Pts',(0.909827729890942,-0.0762225747374255,
0.659680317203144));
#18853=CARTESIAN_POINT('Ctrl Pts',(0.907004864562642,-0.0928409665394228,
0.663576540841106));
#18854=CARTESIAN_POINT('Ctrl Pts',(0.895234408667242,-0.144299303100741,
0.679480524217551));
#18855=CARTESIAN_POINT('Ctrl Pts',(0.882797231409153,-0.177024326825049,
0.695831250979106));
#18856=CARTESIAN_POINT('Ctrl Pts',(0.854332839576145,-0.227269801620064,
0.73042219438957));
#18857=CARTESIAN_POINT('Ctrl Pts',(0.834863020612702,-0.251265615809407,
0.752807465209441));
#18858=CARTESIAN_POINT('Ctrl Pts',(0.800439809856111,-0.279889827963178,
0.789147407129766));
#18859=CARTESIAN_POINT('Ctrl Pts',(0.781998747691871,-0.290879136862659,
0.80756613568454));
#18860=CARTESIAN_POINT('Ctrl Pts',(0.742239891936898,-0.305251990234487,
0.844254137480382));
#18861=CARTESIAN_POINT('Ctrl Pts',(0.720906778729541,-0.308638795020976,
0.862505527716294));
#18862=CARTESIAN_POINT('Ctrl Pts',(0.680463863683392,-0.308638795020976,
0.894757676234429));
#18863=CARTESIAN_POINT('Ctrl Pts',(0.657923009631182,-0.305251990234488,
0.91149460735272));
#18864=CARTESIAN_POINT('Ctrl Pts',(0.613307674922609,-0.290879136862659,
0.942092777160053));
#18865=CARTESIAN_POINT('Ctrl Pts',(0.591247219971725,-0.279889827963178,
0.955972930713954));
#18866=CARTESIAN_POINT('Ctrl Pts',(0.548158511259202,-0.251265615809407,
0.981446681891443));
#18867=CARTESIAN_POINT('Ctrl Pts',(0.522002043615455,-0.227269801620063,
0.995447160474328));
#18868=CARTESIAN_POINT('Ctrl Pts',(0.481944444320713,-0.177024326825049,
1.01550068154148));
#18869=CARTESIAN_POINT('Ctrl Pts',(0.463236132117164,-0.14429930310074,
1.0239876538093));
#18870=CARTESIAN_POINT('Ctrl Pts',(0.445111721969657,-0.0928409665394226,
1.03192403056628));
#18871=CARTESIAN_POINT('Ctrl Pts',(0.440685038163619,-0.0762225747374254,
1.03380912944435));
#18872=CARTESIAN_POINT('Ctrl Pts',(0.437601487681056,-0.05953,1.03511272300331));
#18873=CARTESIAN_POINT('Origin',(0.685838782044607,-0.05953,0.860014630714833));
#18874=CARTESIAN_POINT('Origin',(0.,-0.208355,0.));
#18875=CARTESIAN_POINT('',(0.0548532617164168,-0.05953,1.12247250791415));
#18876=CARTESIAN_POINT('Origin',(0.,-0.05953,0.));
#18877=CARTESIAN_POINT('',(-0.536443649899848,-0.05953,0.987512846410683));
#18878=CARTESIAN_POINT('Ctrl Pts',(0.0548532617164173,-0.0595300000000001,
1.12247250791414));
#18879=CARTESIAN_POINT('Ctrl Pts',(0.05150947068137,-0.0762225747374254,
1.12263591311425));
#18880=CARTESIAN_POINT('Ctrl Pts',(0.0467032526342597,-0.0928409665394227,
1.12285816383385));
#18881=CARTESIAN_POINT('Ctrl Pts',(0.0269302585198975,-0.144299303100741,
1.12357162229597));
#18882=CARTESIAN_POINT('Ctrl Pts',(0.006392292392153,-0.177024326825049,
1.12404235695137));
#18883=CARTESIAN_POINT('Ctrl Pts',(-0.0383992541984087,-0.227269801620063,
1.12335509974011));
#18884=CARTESIAN_POINT('Ctrl Pts',(-0.0680399972366993,-0.251265615809407,
1.12208997038458));
#18885=CARTESIAN_POINT('Ctrl Pts',(-0.117914228755037,-0.279889827963178,
1.1178344036749));
#18886=CARTESIAN_POINT('Ctrl Pts',(-0.14381238480104,-0.290879136862659,
1.11490049012186));
#18887=CARTESIAN_POINT('Ctrl Pts',(-0.19728546073067,-0.305251990234488,
1.10669035995599));
#18888=CARTESIAN_POINT('Ctrl Pts',(-0.224855950742601,-0.308638795020976,
1.10139101611326));
#18889=CARTESIAN_POINT('Ctrl Pts',(-0.275287440920027,-0.308638795020976,
1.0898803575765));
#18890=CARTESIAN_POINT('Ctrl Pts',(-0.302426893214945,-0.305251990234488,
1.08269251410343));
#18891=CARTESIAN_POINT('Ctrl Pts',(-0.35416671187353,-0.290879136862659,
1.06688848765783));
#18892=CARTESIAN_POINT('Ctrl Pts',(-0.3787731215897,-0.279889827963178,
1.05829506364875));
#18893=CARTESIAN_POINT('Ctrl Pts',(-0.425554672694338,-0.251265615809407,
1.04048957871266));
#18894=CARTESIAN_POINT('Ctrl Pts',(-0.452808978448581,-0.227269801620063,
1.02876878445619));
#18895=CARTESIAN_POINT('Ctrl Pts',(-0.493462957200432,-0.177024326825049,
1.0099536580922));
#18896=CARTESIAN_POINT('Ctrl Pts',(-0.511762781179148,-0.14429930310074,
1.00061845128527));
#18897=CARTESIAN_POINT('Ctrl Pts',(-0.529268075276157,-0.0928409665394226,
0.991396466802468));
#18898=CARTESIAN_POINT('Ctrl Pts',(-0.533501897135713,-0.0762225747374254,
0.989110885965947));
#18899=CARTESIAN_POINT('Ctrl Pts',(-0.536443649899848,-0.0595300000000001,
0.987512846410683));
#18900=CARTESIAN_POINT('',(-0.843383895613249,-0.05953,0.742736168477219));
#18901=CARTESIAN_POINT('Origin',(0.,-0.05953,0.));
#18902=CARTESIAN_POINT('',(-1.10653577764992,-0.05953,0.196295654879792));
#18903=CARTESIAN_POINT('Ctrl Pts',(-0.843383895613249,-0.0595300000000001,
0.742736168477219));
#18904=CARTESIAN_POINT('Ctrl Pts',(-0.84559647055299,-0.0762225747374255,
0.740223768851062));
#18905=CARTESIAN_POINT('Ctrl Pts',(-0.848766861100456,-0.0928409665394227,
0.736604687327351));
#18906=CARTESIAN_POINT('Ctrl Pts',(-0.861652925570091,-0.144299303100741,
0.721590372101268));
#18907=CARTESIAN_POINT('Ctrl Pts',(-0.87482617317514,-0.177024326825049,
0.705826641853758));
#18908=CARTESIAN_POINT('Ctrl Pts',(-0.902215926359523,-0.227269801620063,
0.670378702718353));
#18909=CARTESIAN_POINT('Ctrl Pts',(-0.919707509403859,-0.251265615809407,
0.646415841396062));
#18910=CARTESIAN_POINT('Ctrl Pts',(-0.947476448101718,-0.279889827963178,
0.604769294586516));
#18911=CARTESIAN_POINT('Ctrl Pts',(-0.961329858300736,-0.290879136862659,
0.582692035672022));
#18912=CARTESIAN_POINT('Ctrl Pts',(-0.988250837578047,-0.305251990234488,
0.535766169015486));
#18913=CARTESIAN_POINT('Ctrl Pts',(-1.00129756308006,-0.308638795020976,
0.510906605094603));
#18914=CARTESIAN_POINT('Ctrl Pts',(-1.02374168767024,-0.308638795020976,
0.46430090015576));
#18915=CARTESIAN_POINT('Ctrl Pts',(-1.03504317708586,-0.305251990234488,
0.438600874831839));
#18916=CARTESIAN_POINT('Ctrl Pts',(-1.05494634094458,-0.290879136862659,
0.388295406390235));
#18917=CARTESIAN_POINT('Ctrl Pts',(-1.06356957703048,-0.279889827963178,
0.363699428370917));
#18918=CARTESIAN_POINT('Ctrl Pts',(-1.0788165083757,-0.251265615809407,
0.316022600643821));
#18919=CARTESIAN_POINT('Ctrl Pts',(-1.08664560412098,-0.227269801620063,
0.287406530683752));
#18920=CARTESIAN_POINT('Ctrl Pts',(-1.09728268713976,-0.177024326825049,
0.243890930799337));
#18921=CARTESIAN_POINT('Ctrl Pts',(-1.10139388218929,-0.144299303100741,
0.22376314604679));
#18922=CARTESIAN_POINT('Ctrl Pts',(-1.10509821673782,-0.0928409665394227,
0.204327142733961));
#18923=CARTESIAN_POINT('Ctrl Pts',(-1.10595102243643,-0.0762225747374254,
0.199591971170104));
#18924=CARTESIAN_POINT('Ctrl Pts',(-1.10653577764992,-0.0595300000000001,
0.196295654879792));
#18925=CARTESIAN_POINT('',(-1.123812,-0.05953,1.37627276864339E-16));
#18926=CARTESIAN_POINT('Origin',(0.,-0.05953,0.));
#18927=CARTESIAN_POINT('',(-1.123812,-0.35718,1.37627276864339E-16));
#18928=CARTESIAN_POINT('',(-1.123812,-0.208355,1.37627276864339E-16));
#18929=CARTESIAN_POINT('Origin',(0.,-0.35718,0.));
#18930=CARTESIAN_POINT('',(-1.10653577764992,-0.05953,-0.196295654879793));
#18931=CARTESIAN_POINT('Origin',(0.,-0.05953,0.));
#18932=CARTESIAN_POINT('',(-0.843383895613249,-0.05953,-0.742736168477219));
#18933=CARTESIAN_POINT('Ctrl Pts',(-1.10653577764992,-0.0595300000000001,
-0.196295654879792));
#18934=CARTESIAN_POINT('Ctrl Pts',(-1.10595102243643,-0.0762225747374255,
-0.199591971170104));
#18935=CARTESIAN_POINT('Ctrl Pts',(-1.10509821673782,-0.0928409665394228,
-0.204327142733962));
#18936=CARTESIAN_POINT('Ctrl Pts',(-1.10139388218929,-0.144299303100741,
-0.22376314604679));
#18937=CARTESIAN_POINT('Ctrl Pts',(-1.09728268713976,-0.177024326825049,
-0.243890930799338));
#18938=CARTESIAN_POINT('Ctrl Pts',(-1.08664560412098,-0.227269801620063,
-0.287406530683753));
#18939=CARTESIAN_POINT('Ctrl Pts',(-1.0788165083757,-0.251265615809407,
-0.316022600643821));
#18940=CARTESIAN_POINT('Ctrl Pts',(-1.06356957703048,-0.279889827963178,
-0.363699428370918));
#18941=CARTESIAN_POINT('Ctrl Pts',(-1.05494634094458,-0.290879136862659,
-0.388295406390235));
#18942=CARTESIAN_POINT('Ctrl Pts',(-1.03504317708586,-0.305251990234488,
-0.438600874831839));
#18943=CARTESIAN_POINT('Ctrl Pts',(-1.02374168767024,-0.308638795020976,
-0.46430090015576));
#18944=CARTESIAN_POINT('Ctrl Pts',(-1.00129756308006,-0.308638795020976,
-0.510906605094603));
#18945=CARTESIAN_POINT('Ctrl Pts',(-0.988250837578047,-0.305251990234488,
-0.535766169015486));
#18946=CARTESIAN_POINT('Ctrl Pts',(-0.961329858300736,-0.290879136862659,
-0.582692035672022));
#18947=CARTESIAN_POINT('Ctrl Pts',(-0.947476448101718,-0.279889827963178,
-0.604769294586516));
#18948=CARTESIAN_POINT('Ctrl Pts',(-0.919707509403859,-0.251265615809407,
-0.646415841396062));
#18949=CARTESIAN_POINT('Ctrl Pts',(-0.902215926359523,-0.227269801620064,
-0.670378702718353));
#18950=CARTESIAN_POINT('Ctrl Pts',(-0.87482617317514,-0.177024326825049,
-0.705826641853758));
#18951=CARTESIAN_POINT('Ctrl Pts',(-0.861652925570091,-0.144299303100741,
-0.721590372101268));
#18952=CARTESIAN_POINT('Ctrl Pts',(-0.848766861100456,-0.0928409665394229,
-0.736604687327351));
#18953=CARTESIAN_POINT('Ctrl Pts',(-0.84559647055299,-0.0762225747374255,
-0.740223768851063));
#18954=CARTESIAN_POINT('Ctrl Pts',(-0.843383895613249,-0.0595300000000001,
-0.742736168477219));
#18955=CARTESIAN_POINT('',(-0.536443649899847,-0.05953,-0.987512846410683));
#18956=CARTESIAN_POINT('Origin',(0.,-0.05953,0.));
#18957=CARTESIAN_POINT('',(0.0548532617164172,-0.05953,-1.12247250791415));
#18958=CARTESIAN_POINT('Ctrl Pts',(-0.536443649899848,-0.0595300000000001,
-0.987512846410683));
#18959=CARTESIAN_POINT('Ctrl Pts',(-0.533501897135712,-0.0762225747374254,
-0.989110885965947));
#18960=CARTESIAN_POINT('Ctrl Pts',(-0.529268075276156,-0.0928409665394227,
-0.991396466802469));
#18961=CARTESIAN_POINT('Ctrl Pts',(-0.511762781179147,-0.144299303100741,
-1.00061845128527));
#18962=CARTESIAN_POINT('Ctrl Pts',(-0.493462957200432,-0.177024326825049,
-1.0099536580922));
#18963=CARTESIAN_POINT('Ctrl Pts',(-0.45280897844858,-0.227269801620063,
-1.02876878445619));
#18964=CARTESIAN_POINT('Ctrl Pts',(-0.425554672694337,-0.251265615809407,
-1.04048957871266));
#18965=CARTESIAN_POINT('Ctrl Pts',(-0.3787731215897,-0.279889827963178,
-1.05829506364875));
#18966=CARTESIAN_POINT('Ctrl Pts',(-0.354166711873529,-0.290879136862659,
-1.06688848765783));
#18967=CARTESIAN_POINT('Ctrl Pts',(-0.302426893214944,-0.305251990234488,
-1.08269251410343));
#18968=CARTESIAN_POINT('Ctrl Pts',(-0.275287440920027,-0.308638795020976,
-1.0898803575765));
#18969=CARTESIAN_POINT('Ctrl Pts',(-0.224855950742601,-0.308638795020976,
-1.10139101611326));
#18970=CARTESIAN_POINT('Ctrl Pts',(-0.19728546073067,-0.305251990234488,
-1.10669035995599));
#18971=CARTESIAN_POINT('Ctrl Pts',(-0.143812384801039,-0.290879136862659,
-1.11490049012186));
#18972=CARTESIAN_POINT('Ctrl Pts',(-0.117914228755037,-0.279889827963178,
-1.1178344036749));
#18973=CARTESIAN_POINT('Ctrl Pts',(-0.0680399972366989,-0.251265615809407,
-1.12208997038458));
#18974=CARTESIAN_POINT('Ctrl Pts',(-0.0383992541984084,-0.227269801620063,
-1.12335509974011));
#18975=CARTESIAN_POINT('Ctrl Pts',(0.00639229239215326,-0.177024326825049,
-1.12404235695137));
#18976=CARTESIAN_POINT('Ctrl Pts',(0.0269302585198977,-0.144299303100741,
-1.12357162229597));
#18977=CARTESIAN_POINT('Ctrl Pts',(0.04670325263426,-0.0928409665394228,
-1.12285816383385));
#18978=CARTESIAN_POINT('Ctrl Pts',(0.0515094706813703,-0.0762225747374255,
-1.12263591311425));
#18979=CARTESIAN_POINT('Ctrl Pts',(0.0548532617164176,-0.0595300000000001,
-1.12247250791414));
#18980=CARTESIAN_POINT('',(0.437601487681057,-0.05953,-1.03511272300331));
#18981=CARTESIAN_POINT('Origin',(0.,-0.05953,0.));
#18982=CARTESIAN_POINT('',(0.911784794170997,-0.05953,-0.656964154625313));
#18983=CARTESIAN_POINT('Ctrl Pts',(0.437601487681056,-0.0595300000000001,
-1.03511272300331));
#18984=CARTESIAN_POINT('Ctrl Pts',(0.440685038163619,-0.0762225747374255,
-1.03380912944435));
#18985=CARTESIAN_POINT('Ctrl Pts',(0.445111721969657,-0.0928409665394228,
-1.03192403056628));
#18986=CARTESIAN_POINT('Ctrl Pts',(0.463236132117164,-0.144299303100741,
-1.0239876538093));
#18987=CARTESIAN_POINT('Ctrl Pts',(0.481944444320713,-0.177024326825049,
-1.01550068154148));
#18988=CARTESIAN_POINT('Ctrl Pts',(0.522002043615455,-0.227269801620064,
-0.995447160474328));
#18989=CARTESIAN_POINT('Ctrl Pts',(0.548158511259203,-0.251265615809407,
-0.981446681891443));
#18990=CARTESIAN_POINT('Ctrl Pts',(0.591247219971725,-0.279889827963178,
-0.955972930713954));
#18991=CARTESIAN_POINT('Ctrl Pts',(0.613307674922609,-0.290879136862659,
-0.942092777160053));
#18992=CARTESIAN_POINT('Ctrl Pts',(0.657923009631182,-0.305251990234487,
-0.91149460735272));
#18993=CARTESIAN_POINT('Ctrl Pts',(0.680463863683393,-0.308638795020976,
-0.894757676234429));
#18994=CARTESIAN_POINT('Ctrl Pts',(0.720906778729542,-0.308638795020976,
-0.862505527716294));
#18995=CARTESIAN_POINT('Ctrl Pts',(0.742239891936899,-0.305251990234488,
-0.844254137480381));
#18996=CARTESIAN_POINT('Ctrl Pts',(0.781998747691872,-0.290879136862659,
-0.80756613568454));
#18997=CARTESIAN_POINT('Ctrl Pts',(0.800439809856112,-0.279889827963178,
-0.789147407129765));
#18998=CARTESIAN_POINT('Ctrl Pts',(0.834863020612702,-0.251265615809407,
-0.752807465209441));
#18999=CARTESIAN_POINT('Ctrl Pts',(0.854332839576145,-0.227269801620064,
-0.73042219438957));
#19000=CARTESIAN_POINT('Ctrl Pts',(0.882797231409153,-0.177024326825049,
-0.695831250979106));
#19001=CARTESIAN_POINT('Ctrl Pts',(0.895234408667242,-0.144299303100741,
-0.679480524217551));
#19002=CARTESIAN_POINT('Ctrl Pts',(0.907004864562642,-0.0928409665394228,
-0.663576540841106));
#19003=CARTESIAN_POINT('Ctrl Pts',(0.909827729890942,-0.0762225747374256,
-0.659680317203144));
#19004=CARTESIAN_POINT('Ctrl Pts',(0.911784794170998,-0.0595300000000001,
-0.656964154625312));
#19005=CARTESIAN_POINT('',(1.08212377959455,-0.05953,-0.303251606722892));
#19006=CARTESIAN_POINT('Origin',(0.,-0.05953,0.));
#19007=CARTESIAN_POINT('',(1.08212377959455,-0.05953,0.303251606722892));
#19008=CARTESIAN_POINT('Ctrl Pts',(1.08212377959455,-0.0595300000000001,
-0.303251606722892));
#19009=CARTESIAN_POINT('Ctrl Pts',(1.0830271513892,-0.0762225747374255,
-0.300028012588062));
#19010=CARTESIAN_POINT('Ctrl Pts',(1.08431331394788,-0.0928409665394228,
-0.2953917518996));
#19011=CARTESIAN_POINT('Ctrl Pts',(1.08940878963422,-0.144299303100741,
-0.276273267473431));
#19012=CARTESIAN_POINT('Ctrl Pts',(1.09443784939331,-0.177024326825049,
-0.256354979351213));
#19013=CARTESIAN_POINT('Ctrl Pts',(1.10373487993589,-0.227269801620064,
-0.212533521233765));
#19014=CARTESIAN_POINT('Ctrl Pts',(1.10909715583869,-0.251265615809407,
-0.183354415742157));
#19015=CARTESIAN_POINT('Ctrl Pts',(1.1160463456491,-0.279889827963178,-0.133783682657561));
#19016=CARTESIAN_POINT('Ctrl Pts',(1.11894887330541,-0.290879136862659,
-0.107881990270302));
#19017=CARTESIAN_POINT('Ctrl Pts',(1.12284346704144,-0.305251990234488,
-0.0539226701638766));
#19018=CARTESIAN_POINT('Ctrl Pts',(1.123812,-0.308638795020976,-0.025864214957475));
#19019=CARTESIAN_POINT('Ctrl Pts',(1.123812,-0.308638795020976,0.025864214957475));
#19020=CARTESIAN_POINT('Ctrl Pts',(1.12284346704144,-0.305251990234488,
0.0539226701638766));
#19021=CARTESIAN_POINT('Ctrl Pts',(1.11894887330541,-0.290879136862659,
0.107881990270302));
#19022=CARTESIAN_POINT('Ctrl Pts',(1.1160463456491,-0.279889827963178,0.133783682657561));
#19023=CARTESIAN_POINT('Ctrl Pts',(1.10909715583869,-0.251265615809407,
0.183354415742157));
#19024=CARTESIAN_POINT('Ctrl Pts',(1.10373487993589,-0.227269801620064,
0.212533521233765));
#19025=CARTESIAN_POINT('Ctrl Pts',(1.09443784939331,-0.177024326825049,
0.256354979351213));
#19026=CARTESIAN_POINT('Ctrl Pts',(1.08940878963422,-0.144299303100741,
0.276273267473431));
#19027=CARTESIAN_POINT('Ctrl Pts',(1.08431331394788,-0.0928409665394228,
0.2953917518996));
#19028=CARTESIAN_POINT('Ctrl Pts',(1.0830271513892,-0.0762225747374255,
0.300028012588062));
#19029=CARTESIAN_POINT('Ctrl Pts',(1.08212377959455,-0.0595300000000001,
0.303251606722892));
#19030=CARTESIAN_POINT('Origin',(0.,-0.05953,0.));
#19031=CARTESIAN_POINT('Origin',(0.,-0.05953,0.));
#19032=CARTESIAN_POINT('',(0.0589974094846122,-0.05953,1.07456964270265));
#19033=CARTESIAN_POINT('Origin',(0.,-0.05953,0.));
#19034=CARTESIAN_POINT('Origin',(-0.244773027351946,-0.05953,1.07242070340001));
#19035=CARTESIAN_POINT('Origin',(-0.244773027351946,0.,1.07242070340001));
#19036=CARTESIAN_POINT('',(-0.519393123750572,-0.05953,0.942555777842682));
#19037=CARTESIAN_POINT('Ctrl Pts',(-0.519393123750572,-0.05953,0.942555777842682));
#19038=CARTESIAN_POINT('Ctrl Pts',(-0.513714466572041,-0.0925528133349865,
0.945684988399766));
#19039=CARTESIAN_POINT('Ctrl Pts',(-0.503136848051455,-0.124911173756694,
0.951483858396181));
#19040=CARTESIAN_POINT('Ctrl Pts',(-0.47593627990192,-0.177924977804098,
0.965323333309091));
#19041=CARTESIAN_POINT('Ctrl Pts',(-0.460931856495794,-0.199697230012983,
0.972669835243841));
#19042=CARTESIAN_POINT('Ctrl Pts',(-0.426157505475872,-0.237895043532788,
0.988400002689705));
#19043=CARTESIAN_POINT('Ctrl Pts',(-0.406380688682952,-0.254319232363049,
0.996771768218699));
#19044=CARTESIAN_POINT('Ctrl Pts',(-0.364750145543744,-0.28018331644634,
1.01272583306292));
#19045=CARTESIAN_POINT('Ctrl Pts',(-0.340838910881557,-0.29104845371857,
1.02112815447116));
#19046=CARTESIAN_POINT('Ctrl Pts',(-0.290495481564827,-0.30527573347708,
1.036574285215));
#19047=CARTESIAN_POINT('Ctrl Pts',(-0.264056468041074,-0.308638795020976,
1.04359501395068));
#19048=CARTESIAN_POINT('Ctrl Pts',(-0.214892249704082,-0.308638795020976,
1.05481642595959));
#19049=CARTESIAN_POINT('Ctrl Pts',(-0.188025341585962,-0.30527573347708,
1.05996242598502));
#19050=CARTESIAN_POINT('Ctrl Pts',(-0.135965654106109,-0.29104845371857,
1.06788913840721));
#19051=CARTESIAN_POINT('Ctrl Pts',(-0.110776745452494,-0.28018331644634,
1.07069360430242));
#19052=CARTESIAN_POINT('Ctrl Pts',(-0.0663467128214646,-0.254319232363049,
1.07438230428002));
#19053=CARTESIAN_POINT('Ctrl Pts',(-0.0448960436540983,-0.237895043532788,
1.07542044338697));
#19054=CARTESIAN_POINT('Ctrl Pts',(-0.00674037211528124,-0.199697230012983,
1.07633607767727));
#19055=CARTESIAN_POINT('Ctrl Pts',(0.00996567398334777,-0.177924977804098,
1.07622728347683));
#19056=CARTESIAN_POINT('Ctrl Pts',(0.0404772621979741,-0.124911173756694,
1.07556023164702));
#19057=CARTESIAN_POINT('Ctrl Pts',(0.0525234025782719,-0.0925528133349865,
1.07492508698591));
#19058=CARTESIAN_POINT('Ctrl Pts',(0.0589974094846124,-0.05953,1.07456964270265));
#19059=CARTESIAN_POINT('Origin',(-0.244773027351946,-0.05953,1.07242070340001));
#19060=CARTESIAN_POINT('Origin',(0.,-0.05953,0.));
#19061=CARTESIAN_POINT('',(-0.803348093619616,-0.05953,0.716109245731214));
#19062=CARTESIAN_POINT('Origin',(0.,-0.05953,0.));
#19063=CARTESIAN_POINT('Origin',(-0.991065754692661,-0.05953,0.477272113029314));
#19064=CARTESIAN_POINT('Origin',(-0.991065754692661,0.,0.477272113029314));
#19065=CARTESIAN_POINT('',(-1.06075609691358,-0.05953,0.181596019242328));
#19066=CARTESIAN_POINT('Ctrl Pts',(-1.06075609691358,-0.05953,0.181596019242328));
#19067=CARTESIAN_POINT('Ctrl Pts',(-1.05966202740332,-0.0925528133349865,
0.187986803072856));
#19068=CARTESIAN_POINT('Ctrl Pts',(-1.05760072925372,-0.124911173756694,
0.199872254546857));
#19069=CARTESIAN_POINT('Ctrl Pts',(-1.05146158959546,-0.177924977804098,
0.22976728653846));
#19070=CARTESIAN_POINT('Ctrl Pts',(-1.04785021111757,-0.199697230012983,
0.246078686169301));
#19071=CARTESIAN_POINT('Ctrl Pts',(-1.03846709802406,-0.237895043532788,
0.283073967563097));
#19072=CARTESIAN_POINT('Ctrl Pts',(-1.03268176429485,-0.254319232363049,
0.303755815985685));
#19073=CARTESIAN_POINT('Ctrl Pts',(-1.01919893537026,-0.28018331644634,
0.346251081972725));
#19074=CARTESIAN_POINT('Ctrl Pts',(-1.01085972381132,-0.29104845371857,
0.370184399726282));
#19075=CARTESIAN_POINT('Ctrl Pts',(-0.99154738033959,-0.30527573347708,
0.419174982698463));
#19076=CARTESIAN_POINT('Ctrl Pts',(-0.980551951791748,-0.308638795020976,
0.444223188605045));
#19077=CARTESIAN_POINT('Ctrl Pts',(-0.958671816228589,-0.308638795020976,
0.489657758261848));
#19078=CARTESIAN_POINT('Ctrl Pts',(-0.945943877838127,-0.30527573347708,
0.51387163140139));
#19079=CARTESIAN_POINT('Ctrl Pts',(-0.91968254693063,-0.29104845371857,
0.559515758398093));
#19080=CARTESIAN_POINT('Ctrl Pts',(-0.906170138993533,-0.28018331644634,
0.580957796077825));
#19081=CARTESIAN_POINT('Ctrl Pts',(-0.8813524085237,-0.254319232363049,
0.617994461173994));
#19082=CARTESIAN_POINT('Ctrl Pts',(-0.868789784891799,-0.237895043532788,
0.635412538795143));
#19083=CARTESIAN_POINT('Ctrl Pts',(-0.845715984518854,-0.199697230012983,
0.66581473268113));
#19084=CARTESIAN_POINT('Ctrl Pts',(-0.835214876415962,-0.177924977804098,
0.678808213394124));
#19085=CARTESIAN_POINT('Ctrl Pts',(-0.815669690204649,-0.124911173756694,
0.702247233627224));
#19086=CARTESIAN_POINT('Ctrl Pts',(-0.807662468433796,-0.0925528133349865,
0.711269279199861));
#19087=CARTESIAN_POINT('Ctrl Pts',(-0.803348093619616,-0.05953,0.716109245731214));
#19088=CARTESIAN_POINT('Origin',(-0.991065754692661,-0.05953,0.477272113029314));
#19089=CARTESIAN_POINT('Origin',(0.,-0.05953,0.));
#19090=CARTESIAN_POINT('',(-1.076188,-0.05953,1.31795018948079E-16));
#19091=CARTESIAN_POINT('Origin',(0.,-0.05953,0.));
#19092=CARTESIAN_POINT('',(-1.06075609691358,-0.05953,-0.181596019242328));
#19093=CARTESIAN_POINT('Origin',(0.,-0.05953,0.));
#19094=CARTESIAN_POINT('Origin',(-0.991065754692661,-0.05953,-0.477272113029314));
#19095=CARTESIAN_POINT('Origin',(-0.991065754692661,0.,-0.477272113029314));
#19096=CARTESIAN_POINT('',(-0.803348093619616,-0.05953,-0.716109245731215));
#19097=CARTESIAN_POINT('Ctrl Pts',(-0.803348093619616,-0.05953,-0.716109245731215));
#19098=CARTESIAN_POINT('Ctrl Pts',(-0.807662468433795,-0.0925528133349865,
-0.711269279199862));
#19099=CARTESIAN_POINT('Ctrl Pts',(-0.815669690204649,-0.124911173756694,
-0.702247233627224));
#19100=CARTESIAN_POINT('Ctrl Pts',(-0.835214876415962,-0.177924977804098,
-0.678808213394124));
#19101=CARTESIAN_POINT('Ctrl Pts',(-0.845715984518854,-0.199697230012983,
-0.66581473268113));
#19102=CARTESIAN_POINT('Ctrl Pts',(-0.868789784891799,-0.237895043532788,
-0.635412538795143));
#19103=CARTESIAN_POINT('Ctrl Pts',(-0.8813524085237,-0.254319232363049,
-0.617994461173994));
#19104=CARTESIAN_POINT('Ctrl Pts',(-0.906170138993533,-0.28018331644634,
-0.580957796077826));
#19105=CARTESIAN_POINT('Ctrl Pts',(-0.91968254693063,-0.29104845371857,
-0.559515758398093));
#19106=CARTESIAN_POINT('Ctrl Pts',(-0.945943877838127,-0.30527573347708,
-0.51387163140139));
#19107=CARTESIAN_POINT('Ctrl Pts',(-0.958671816228589,-0.308638795020976,
-0.489657758261848));
#19108=CARTESIAN_POINT('Ctrl Pts',(-0.980551951791748,-0.308638795020976,
-0.444223188605045));
#19109=CARTESIAN_POINT('Ctrl Pts',(-0.99154738033959,-0.30527573347708,
-0.419174982698463));
#19110=CARTESIAN_POINT('Ctrl Pts',(-1.01085972381132,-0.29104845371857,
-0.370184399726282));
#19111=CARTESIAN_POINT('Ctrl Pts',(-1.01919893537026,-0.28018331644634,
-0.346251081972725));
#19112=CARTESIAN_POINT('Ctrl Pts',(-1.03268176429485,-0.254319232363049,
-0.303755815985685));
#19113=CARTESIAN_POINT('Ctrl Pts',(-1.03846709802406,-0.237895043532788,
-0.283073967563097));
#19114=CARTESIAN_POINT('Ctrl Pts',(-1.04785021111757,-0.199697230012983,
-0.246078686169302));
#19115=CARTESIAN_POINT('Ctrl Pts',(-1.05146158959546,-0.177924977804098,
-0.229767286538461));
#19116=CARTESIAN_POINT('Ctrl Pts',(-1.05760072925372,-0.124911173756694,
-0.199872254546858));
#19117=CARTESIAN_POINT('Ctrl Pts',(-1.05966202740332,-0.0925528133349864,
-0.187986803072857));
#19118=CARTESIAN_POINT('Ctrl Pts',(-1.06075609691358,-0.05953,-0.181596019242328));
#19119=CARTESIAN_POINT('Origin',(-0.991065754692661,-0.05953,-0.477272113029314));
#19120=CARTESIAN_POINT('Origin',(0.,-0.05953,0.));
#19121=CARTESIAN_POINT('',(-0.519393123750572,-0.05953,-0.942555777842682));
#19122=CARTESIAN_POINT('Origin',(0.,-0.05953,0.));
#19123=CARTESIAN_POINT('Origin',(-0.244773027351946,-0.05953,-1.07242070340001));
#19124=CARTESIAN_POINT('Origin',(-0.244773027351946,0.,-1.07242070340001));
#19125=CARTESIAN_POINT('',(0.0589974094846125,-0.05953,-1.07456964270265));
#19126=CARTESIAN_POINT('Ctrl Pts',(0.0589974094846127,-0.05953,-1.07456964270265));
#19127=CARTESIAN_POINT('Ctrl Pts',(0.0525234025782722,-0.0925528133349865,
-1.07492508698591));
#19128=CARTESIAN_POINT('Ctrl Pts',(0.0404772621979744,-0.124911173756694,
-1.07556023164702));
#19129=CARTESIAN_POINT('Ctrl Pts',(0.0099656739833481,-0.177924977804098,
-1.07622728347683));
#19130=CARTESIAN_POINT('Ctrl Pts',(-0.00674037211528096,-0.199697230012983,
-1.07633607767727));
#19131=CARTESIAN_POINT('Ctrl Pts',(-0.044896043654098,-0.237895043532788,
-1.07542044338697));
#19132=CARTESIAN_POINT('Ctrl Pts',(-0.0663467128214644,-0.254319232363049,
-1.07438230428002));
#19133=CARTESIAN_POINT('Ctrl Pts',(-0.110776745452493,-0.28018331644634,
-1.07069360430242));
#19134=CARTESIAN_POINT('Ctrl Pts',(-0.135965654106109,-0.29104845371857,
-1.06788913840721));
#19135=CARTESIAN_POINT('Ctrl Pts',(-0.188025341585962,-0.30527573347708,
-1.05996242598502));
#19136=CARTESIAN_POINT('Ctrl Pts',(-0.214892249704082,-0.308638795020976,
-1.05481642595959));
#19137=CARTESIAN_POINT('Ctrl Pts',(-0.264056468041074,-0.308638795020976,
-1.04359501395068));
#19138=CARTESIAN_POINT('Ctrl Pts',(-0.290495481564827,-0.30527573347708,
-1.036574285215));
#19139=CARTESIAN_POINT('Ctrl Pts',(-0.340838910881557,-0.291048453718569,
-1.02112815447116));
#19140=CARTESIAN_POINT('Ctrl Pts',(-0.364750145543744,-0.28018331644634,
-1.01272583306292));
#19141=CARTESIAN_POINT('Ctrl Pts',(-0.406380688682952,-0.254319232363049,
-0.996771768218699));
#19142=CARTESIAN_POINT('Ctrl Pts',(-0.426157505475872,-0.237895043532788,
-0.988400002689705));
#19143=CARTESIAN_POINT('Ctrl Pts',(-0.460931856495794,-0.199697230012983,
-0.972669835243841));
#19144=CARTESIAN_POINT('Ctrl Pts',(-0.475936279901919,-0.177924977804098,
-0.965323333309091));
#19145=CARTESIAN_POINT('Ctrl Pts',(-0.503136848051454,-0.124911173756694,
-0.951483858396181));
#19146=CARTESIAN_POINT('Ctrl Pts',(-0.513714466572041,-0.0925528133349865,
-0.945684988399766));
#19147=CARTESIAN_POINT('Ctrl Pts',(-0.519393123750572,-0.05953,-0.942555777842682));
#19148=CARTESIAN_POINT('Origin',(-0.244773027351946,-0.05953,-1.07242070340001));
#19149=CARTESIAN_POINT('Origin',(0.,-0.05953,0.));
#19150=CARTESIAN_POINT('',(0.413083465285518,-0.05953,-0.993751811093549));
#19151=CARTESIAN_POINT('Origin',(0.,-0.05953,0.));
#19152=CARTESIAN_POINT('Origin',(0.685838782044607,-0.05953,-0.860014630714833));
#19153=CARTESIAN_POINT('Origin',(0.685838782044607,0.,-0.860014630714833));
#19154=CARTESIAN_POINT('',(0.876916659919095,-0.05953,-0.623857181492959));
#19155=CARTESIAN_POINT('Ctrl Pts',(0.876916659919095,-0.05953,-0.623857181492958));
#19156=CARTESIAN_POINT('Ctrl Pts',(0.873158080166742,-0.0925528133349865,
-0.62914037979579));
#19157=CARTESIAN_POINT('Ctrl Pts',(0.866144010579847,-0.124911173756694,
-0.638954437806245));
#19158=CARTESIAN_POINT('Ctrl Pts',(0.847641868610495,-0.177924977804098,
-0.663225258065736));
#19159=CARTESIAN_POINT('Ctrl Pts',(0.837310877969633,-0.199697230012983,
-0.676354402927683));
#19160=CARTESIAN_POINT('Ctrl Pts',(0.81280533416753,-0.237895043532788,
-0.705614819529209));
#19161=CARTESIAN_POINT('Ctrl Pts',(0.798619410861634,-0.254319232363049,
-0.721738358858166));
#19162=CARTESIAN_POINT('Ctrl Pts',(0.768033796848072,-0.28018331644634,
-0.754175290318038));
#19163=CARTESIAN_POINT('Ctrl Pts',(0.750136149454208,-0.29104845371857,
-0.772120216227122));
#19164=CARTESIAN_POINT('Ctrl Pts',(0.711480111898423,-0.30527573347708,
-0.807879894508811));
#19165=CARTESIAN_POINT('Ctrl Pts',(0.690705563850638,-0.308638795020976,
-0.825676810575913));
#19166=CARTESIAN_POINT('Ctrl Pts',(0.651278921914856,-0.308638795020976,
-0.857118508332695));
#19167=CARTESIAN_POINT('Ctrl Pts',(0.629305439856167,-0.30527573347708,
-0.873412008702649));
#19168=CARTESIAN_POINT('Ctrl Pts',(0.585840553788742,-0.29104845371857,
-0.903141581680914));
#19169=CARTESIAN_POINT('Ctrl Pts',(0.564362943424239,-0.28018331644634,
-0.916597376014514));
#19170=CARTESIAN_POINT('Ctrl Pts',(0.525933334162556,-0.254319232363049,
-0.939198248544427));
#19171=CARTESIAN_POINT('Ctrl Pts',(0.507057380724533,-0.237895043532788,
-0.949440676105255));
#19172=CARTESIAN_POINT('Ctrl Pts',(0.473077587363686,-0.199697230012983,
-0.966820759530997));
#19173=CARTESIAN_POINT('Ctrl Pts',(0.457978755888596,-0.177924977804098,
-0.973971221090534));
#19174=CARTESIAN_POINT('Ctrl Pts',(0.430199341854858,-0.124911173756694,
-0.986608710139579));
#19175=CARTESIAN_POINT('Ctrl Pts',(0.419070565453384,-0.0925528133349865,
-0.991263089003441));
#19176=CARTESIAN_POINT('Ctrl Pts',(0.413083465285518,-0.05953,-0.993751811093549));
#19177=CARTESIAN_POINT('Origin',(0.685838782044607,-0.05953,-0.860014630714833));
#19178=CARTESIAN_POINT('Origin',(0.,-0.208355,0.));
#19179=CARTESIAN_POINT('',(-1.076188,-0.35718,1.31795018948079E-16));
#19180=CARTESIAN_POINT('Origin',(0.,-0.35718,0.));
#19181=CARTESIAN_POINT('',(-1.076188,-0.208355,1.31795018948079E-16));
#19182=CARTESIAN_POINT('',(1.03449977959455,-0.05953,0.296632461748266));
#19183=CARTESIAN_POINT('Origin',(0.,-0.05953,0.));
#19184=CARTESIAN_POINT('',(1.03449977959455,-0.05953,-0.296632461748266));
#19185=CARTESIAN_POINT('Ctrl Pts',(1.03449977959455,-0.05953,0.296632461748267));
#19186=CARTESIAN_POINT('Ctrl Pts',(1.03628691421076,-0.0925528133349865,
0.290399865505497));
#19187=CARTESIAN_POINT('Ctrl Pts',(1.03958665287714,-0.124911173756694,
0.278797079997872));
#19188=CARTESIAN_POINT('Ctrl Pts',(1.0470264474309,-0.177924977804098,0.249198913998601));
#19189=CARTESIAN_POINT('Ctrl Pts',(1.05084995891418,-0.199697230012983,
0.232935932341942));
#19190=CARTESIAN_POINT('Ctrl Pts',(1.05844771715377,-0.237895043532788,
0.195533155353269));
#19191=CARTESIAN_POINT('Ctrl Pts',(1.06220882929878,-0.254319232363049,
0.17438929156337));
#19192=CARTESIAN_POINT('Ctrl Pts',(1.06849922508772,-0.28018331644634,0.130252399648131));
#19193=CARTESIAN_POINT('Ctrl Pts',(1.07137013248666,-0.29104845371857,0.105070977154072));
#19194=CARTESIAN_POINT('Ctrl Pts',(1.07522652957392,-0.30527573347708,0.0525526752791107));
#19195=CARTESIAN_POINT('Ctrl Pts',(1.076188,-0.308638795020976,0.025214283908933));
#19196=CARTESIAN_POINT('Ctrl Pts',(1.076188,-0.308638795020976,-0.025214283908933));
#19197=CARTESIAN_POINT('Ctrl Pts',(1.07522652957392,-0.30527573347708,-0.0525526752791107));
#19198=CARTESIAN_POINT('Ctrl Pts',(1.07137013248666,-0.29104845371857,-0.105070977154072));
#19199=CARTESIAN_POINT('Ctrl Pts',(1.06849922508772,-0.28018331644634,-0.130252399648131));
#19200=CARTESIAN_POINT('Ctrl Pts',(1.06220882929878,-0.254319232363049,
-0.17438929156337));
#19201=CARTESIAN_POINT('Ctrl Pts',(1.05844771715377,-0.237895043532788,
-0.195533155353269));
#19202=CARTESIAN_POINT('Ctrl Pts',(1.05084995891418,-0.199697230012983,
-0.232935932341942));
#19203=CARTESIAN_POINT('Ctrl Pts',(1.0470264474309,-0.177924977804098,-0.249198913998601));
#19204=CARTESIAN_POINT('Ctrl Pts',(1.03958665287714,-0.124911173756694,
-0.278797079997872));
#19205=CARTESIAN_POINT('Ctrl Pts',(1.03628691421076,-0.0925528133349865,
-0.290399865505497));
#19206=CARTESIAN_POINT('Ctrl Pts',(1.03449977959455,-0.05953,-0.296632461748267));
#19207=CARTESIAN_POINT('Origin',(0.,-0.05953,0.));
#19208=CARTESIAN_POINT('Origin',(0.,-0.05953,0.));
#19209=CARTESIAN_POINT('Origin',(1.1,-0.05953,0.));
#19210=CARTESIAN_POINT('Origin',(1.1,0.,0.));
#19211=CARTESIAN_POINT('Origin',(1.1,-0.05953,0.));
#19212=CARTESIAN_POINT('Origin',(0.,-0.35718,0.));
#19213=CARTESIAN_POINT('Origin',(0.,-0.05953,0.));
#32676=UNCERTAINTY_MEASURE_WITH_UNIT(LENGTH_MEASURE(0.001),#32752,
'DISTANCE_ACCURACY_VALUE',
'Maximum model space distance between geometric entities at asserted c
onnectivities');
#32702=UNCERTAINTY_MEASURE_WITH_UNIT(LENGTH_MEASURE(0.001),#32752,
'DISTANCE_ACCURACY_VALUE',
'Maximum model space distance between geometric entities at asserted c
onnectivities');
#32725=(
GEOMETRIC_REPRESENTATION_CONTEXT(3)
GLOBAL_UNCERTAINTY_ASSIGNED_CONTEXT((#32676))
GLOBAL_UNIT_ASSIGNED_CONTEXT((#32752,#32754,#32755))
REPRESENTATION_CONTEXT('','3D')
);
#32751=(
GEOMETRIC_REPRESENTATION_CONTEXT(3)
GLOBAL_UNCERTAINTY_ASSIGNED_CONTEXT((#32702))
GLOBAL_UNIT_ASSIGNED_CONTEXT((#32752,#32754,#32755))
REPRESENTATION_CONTEXT('','3D')
);
#32752=(
LENGTH_UNIT()
NAMED_UNIT(*)
SI_UNIT(.CENTI.,.METRE.)
);
#32754=(
NAMED_UNIT(*)
PLANE_ANGLE_UNIT()
SI_UNIT($,.RADIAN.)
);
#32755=(
NAMED_UNIT(*)
SI_UNIT($,.STERADIAN.)
SOLID_ANGLE_UNIT()
);
#32778=SHAPE_DEFINITION_REPRESENTATION(#32826,#32951);
#32826=PRODUCT_DEFINITION_SHAPE('',$,#33000);
#32951=SHAPE_REPRESENTATION('',(#13470),#32725);
#32977=PRODUCT_DEFINITION_CONTEXT('part definition',#33123,'design');
#33000=PRODUCT_DEFINITION('Cage','Cage',#33048,#32977);
#33048=PRODUCT_DEFINITION_FORMATION('',$,#33147);
#33123=APPLICATION_CONTEXT(
'Core Data for Automotive Mechanical Design Process');
#33124=PRODUCT_CONTEXT('part definition',#33123,'mechanical');
#33147=PRODUCT('Cage','Cage','Cage',(#33124));
#33236=COLOUR_RGB('Grey',0.48,0.52,0.57);
#33237=FILL_AREA_STYLE_COLOUR('',#33236);
#33238=FILL_AREA_STYLE('',(#33237));
#33239=SURFACE_STYLE_FILL_AREA(#33238);
#33240=SURFACE_SIDE_STYLE('',(#33239));
#33241=SURFACE_STYLE_USAGE(.BOTH.,#33240);
#33242=PRESENTATION_STYLE_ASSIGNMENT((#33241));
ENDSEC;
END-ISO-10303-21;
